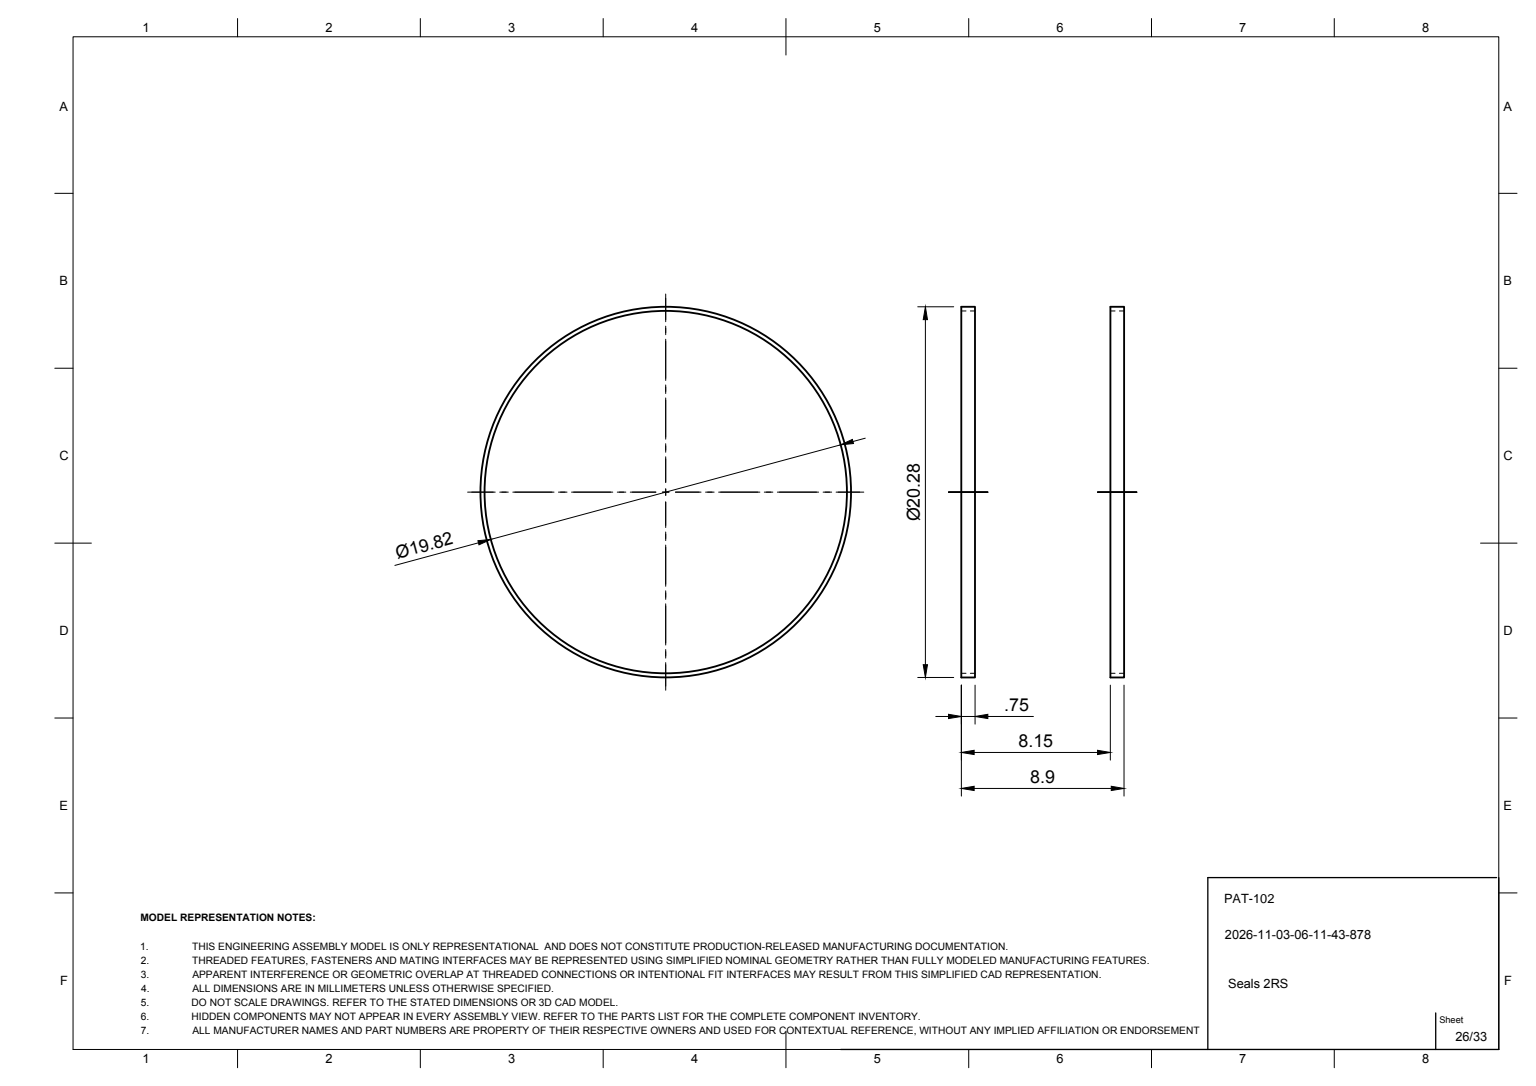
ISO-10303-21;
HEADER;
/* Generated by software containing ST-Developer
 * from STEP Tools, Inc. (www.steptools.com) 
 */

FILE_DESCRIPTION(
/* description */ ('Swing-away clamp arm'),
/* implementation_level */ '2;1');

FILE_NAME(
/* name */ 'Seals 2RS.step',
/* time_stamp */ '2026-10-28T03:26:03-07:00',
/* author */ (''),
/* organization */ (''),
/* preprocessor_version */ 'ST-DEVELOPER v20.2',
/* originating_system */ 'Autodesk Translation Framework v15.17.0.0',
/* authorisation */ '');

FILE_SCHEMA (('AUTOMOTIVE_DESIGN { 1 0 10303 214 3 1 1 }'));
ENDSEC;

DATA;
#10=MECHANICAL_DESIGN_GEOMETRIC_PRESENTATION_REPRESENTATION('',(#318,#319),#10627);
#259=SHAPE_REPRESENTATION_RELATIONSHIP('SRR','None',#10759,#285);
#285=ADVANCED_BREP_SHAPE_REPRESENTATION('',(#351,#352),#10618);
#318=STYLED_ITEM('',(#10965),#351);
#319=STYLED_ITEM('',(#10965),#352);
#351=MANIFOLD_SOLID_BREP('Body1',#4925);
#352=MANIFOLD_SOLID_BREP('Body2',#4926);
#437=FACE_BOUND('',#1253,.T.);
#438=FACE_BOUND('',#1256,.T.);
#439=FACE_BOUND('',#1259,.T.);
#440=FACE_BOUND('',#1262,.T.);
#591=PLANE('',#5692);
#592=PLANE('',#5697);
#593=PLANE('',#5700);
#594=PLANE('',#5705);
#866=FACE_OUTER_BOUND('',#1252,.T.);
#867=FACE_OUTER_BOUND('',#1254,.T.);
#868=FACE_OUTER_BOUND('',#1255,.T.);
#869=FACE_OUTER_BOUND('',#1257,.T.);
#870=FACE_OUTER_BOUND('',#1258,.T.);
#871=FACE_OUTER_BOUND('',#1260,.T.);
#872=FACE_OUTER_BOUND('',#1261,.T.);
#873=FACE_OUTER_BOUND('',#1263,.T.);
#1252=EDGE_LOOP('',(#4229));
#1253=EDGE_LOOP('',(#4230));
#1254=EDGE_LOOP('',(#4231,#4232,#4233,#4234));
#1255=EDGE_LOOP('',(#4235));
#1256=EDGE_LOOP('',(#4236));
#1257=EDGE_LOOP('',(#4237,#4238,#4239,#4240));
#1258=EDGE_LOOP('',(#4241));
#1259=EDGE_LOOP('',(#4242));
#1260=EDGE_LOOP('',(#4243,#4244,#4245,#4246));
#1261=EDGE_LOOP('',(#4247));
#1262=EDGE_LOOP('',(#4248));
#1263=EDGE_LOOP('',(#4249,#4250,#4251,#4252));
#1598=LINE('',#10232,#1920);
#1599=LINE('',#10237,#1921);
#1600=LINE('',#10246,#1922);
#1601=LINE('',#10251,#1923);
#1920=VECTOR('',#7065,1.013815);
#1921=VECTOR('',#7072,0.991185);
#1922=VECTOR('',#7083,1.013815);
#1923=VECTOR('',#7090,0.991185);
#2203=CIRCLE('',#5693,1.013815);
#2204=CIRCLE('',#5694,0.991185);
#2205=CIRCLE('',#5696,1.013815);
#2206=CIRCLE('',#5698,0.991185);
#2207=CIRCLE('',#5701,1.013815);
#2208=CIRCLE('',#5702,0.991185);
#2209=CIRCLE('',#5704,1.013815);
#2210=CIRCLE('',#5706,0.991185);
#2586=VERTEX_POINT('',#10225);
#2587=VERTEX_POINT('',#10227);
#2588=VERTEX_POINT('',#10230);
#2589=VERTEX_POINT('',#10234);
#2590=VERTEX_POINT('',#10239);
#2591=VERTEX_POINT('',#10241);
#2592=VERTEX_POINT('',#10244);
#2593=VERTEX_POINT('',#10248);
#3147=EDGE_CURVE('',#2586,#2586,#2203,.T.);
#3148=EDGE_CURVE('',#2587,#2587,#2204,.T.);
#3149=EDGE_CURVE('',#2588,#2588,#2205,.T.);
#3150=EDGE_CURVE('',#2588,#2586,#1598,.T.);
#3151=EDGE_CURVE('',#2589,#2589,#2206,.T.);
#3152=EDGE_CURVE('',#2589,#2587,#1599,.T.);
#3153=EDGE_CURVE('',#2590,#2590,#2207,.T.);
#3154=EDGE_CURVE('',#2591,#2591,#2208,.T.);
#3155=EDGE_CURVE('',#2592,#2592,#2209,.T.);
#3156=EDGE_CURVE('',#2592,#2590,#1600,.T.);
#3157=EDGE_CURVE('',#2593,#2593,#2210,.T.);
#3158=EDGE_CURVE('',#2593,#2591,#1601,.T.);
#4229=ORIENTED_EDGE('',*,*,#3147,.F.);
#4230=ORIENTED_EDGE('',*,*,#3148,.T.);
#4231=ORIENTED_EDGE('',*,*,#3149,.F.);
#4232=ORIENTED_EDGE('',*,*,#3150,.T.);
#4233=ORIENTED_EDGE('',*,*,#3147,.T.);
#4234=ORIENTED_EDGE('',*,*,#3150,.F.);
#4235=ORIENTED_EDGE('',*,*,#3149,.T.);
#4236=ORIENTED_EDGE('',*,*,#3151,.F.);
#4237=ORIENTED_EDGE('',*,*,#3151,.T.);
#4238=ORIENTED_EDGE('',*,*,#3152,.T.);
#4239=ORIENTED_EDGE('',*,*,#3148,.F.);
#4240=ORIENTED_EDGE('',*,*,#3152,.F.);
#4241=ORIENTED_EDGE('',*,*,#3153,.F.);
#4242=ORIENTED_EDGE('',*,*,#3154,.T.);
#4243=ORIENTED_EDGE('',*,*,#3155,.F.);
#4244=ORIENTED_EDGE('',*,*,#3156,.T.);
#4245=ORIENTED_EDGE('',*,*,#3153,.T.);
#4246=ORIENTED_EDGE('',*,*,#3156,.F.);
#4247=ORIENTED_EDGE('',*,*,#3155,.T.);
#4248=ORIENTED_EDGE('',*,*,#3157,.F.);
#4249=ORIENTED_EDGE('',*,*,#3157,.T.);
#4250=ORIENTED_EDGE('',*,*,#3158,.T.);
#4251=ORIENTED_EDGE('',*,*,#3154,.F.);
#4252=ORIENTED_EDGE('',*,*,#3158,.F.);
#4567=CYLINDRICAL_SURFACE('',#5695,1.013815);
#4568=CYLINDRICAL_SURFACE('',#5699,0.991185);
#4569=CYLINDRICAL_SURFACE('',#5703,1.013815);
#4570=CYLINDRICAL_SURFACE('',#5707,0.991185);
#4821=ADVANCED_FACE('',(#866,#437),#591,.T.);
#4822=ADVANCED_FACE('',(#867),#4567,.T.);
#4823=ADVANCED_FACE('',(#868,#438),#592,.T.);
#4824=ADVANCED_FACE('',(#869),#4568,.F.);
#4825=ADVANCED_FACE('',(#870,#439),#593,.T.);
#4826=ADVANCED_FACE('',(#871),#4569,.T.);
#4827=ADVANCED_FACE('',(#872,#440),#594,.T.);
#4828=ADVANCED_FACE('',(#873),#4570,.F.);
#4925=CLOSED_SHELL('',(#4821,#4822,#4823,#4824));
#4926=CLOSED_SHELL('',(#4825,#4826,#4827,#4828));
#5691=AXIS2_PLACEMENT_3D('',#10223,#7053,#7054);
#5692=AXIS2_PLACEMENT_3D('',#10224,#7055,#7056);
#5693=AXIS2_PLACEMENT_3D('',#10226,#7057,#7058);
#5694=AXIS2_PLACEMENT_3D('',#10228,#7059,#7060);
#5695=AXIS2_PLACEMENT_3D('',#10229,#7061,#7062);
#5696=AXIS2_PLACEMENT_3D('',#10231,#7063,#7064);
#5697=AXIS2_PLACEMENT_3D('',#10233,#7066,#7067);
#5698=AXIS2_PLACEMENT_3D('',#10235,#7068,#7069);
#5699=AXIS2_PLACEMENT_3D('',#10236,#7070,#7071);
#5700=AXIS2_PLACEMENT_3D('',#10238,#7073,#7074);
#5701=AXIS2_PLACEMENT_3D('',#10240,#7075,#7076);
#5702=AXIS2_PLACEMENT_3D('',#10242,#7077,#7078);
#5703=AXIS2_PLACEMENT_3D('',#10243,#7079,#7080);
#5704=AXIS2_PLACEMENT_3D('',#10245,#7081,#7082);
#5705=AXIS2_PLACEMENT_3D('',#10247,#7084,#7085);
#5706=AXIS2_PLACEMENT_3D('',#10249,#7086,#7087);
#5707=AXIS2_PLACEMENT_3D('',#10250,#7088,#7089);
#7053=DIRECTION('axis',(0.,0.,1.));
#7054=DIRECTION('refdir',(1.,0.,0.));
#7055=DIRECTION('center_axis',(0.,1.,0.));
#7056=DIRECTION('ref_axis',(0.,0.,1.));
#7057=DIRECTION('center_axis',(0.,-1.,0.));
#7058=DIRECTION('ref_axis',(1.,0.,0.));
#7059=DIRECTION('center_axis',(0.,-1.,0.));
#7060=DIRECTION('ref_axis',(1.,0.,0.));
#7061=DIRECTION('center_axis',(0.,-1.,0.));
#7062=DIRECTION('ref_axis',(1.,0.,0.));
#7063=DIRECTION('center_axis',(0.,-1.,0.));
#7064=DIRECTION('ref_axis',(1.,0.,0.));
#7065=DIRECTION('',(0.,1.,0.));
#7066=DIRECTION('center_axis',(0.,-1.,0.));
#7067=DIRECTION('ref_axis',(0.,0.,-1.));
#7068=DIRECTION('center_axis',(0.,-1.,0.));
#7069=DIRECTION('ref_axis',(1.,0.,0.));
#7070=DIRECTION('center_axis',(0.,-1.,0.));
#7071=DIRECTION('ref_axis',(1.,0.,0.));
#7072=DIRECTION('',(0.,1.,0.));
#7073=DIRECTION('center_axis',(0.,1.,0.));
#7074=DIRECTION('ref_axis',(0.,0.,1.));
#7075=DIRECTION('center_axis',(0.,-1.,0.));
#7076=DIRECTION('ref_axis',(1.,0.,0.));
#7077=DIRECTION('center_axis',(0.,-1.,0.));
#7078=DIRECTION('ref_axis',(1.,0.,0.));
#7079=DIRECTION('center_axis',(0.,-1.,0.));
#7080=DIRECTION('ref_axis',(1.,0.,0.));
#7081=DIRECTION('center_axis',(0.,-1.,0.));
#7082=DIRECTION('ref_axis',(1.,0.,0.));
#7083=DIRECTION('',(0.,1.,0.));
#7084=DIRECTION('center_axis',(0.,-1.,0.));
#7085=DIRECTION('ref_axis',(0.,0.,-1.));
#7086=DIRECTION('center_axis',(0.,-1.,0.));
#7087=DIRECTION('ref_axis',(1.,0.,0.));
#7088=DIRECTION('center_axis',(0.,-1.,0.));
#7089=DIRECTION('ref_axis',(1.,0.,0.));
#7090=DIRECTION('',(0.,1.,0.));
#10223=CARTESIAN_POINT('',(0.,0.,0.));
#10224=CARTESIAN_POINT('Origin',(1.013815,0.445,0.));
#10225=CARTESIAN_POINT('',(-1.013815,0.445,-1.24156529467757E-16));
#10226=CARTESIAN_POINT('Origin',(0.,0.445,0.));
#10227=CARTESIAN_POINT('',(-0.991185,0.445,-1.21385153761287E-16));
#10228=CARTESIAN_POINT('Origin',(0.,0.445,0.));
#10229=CARTESIAN_POINT('Origin',(0.,0.4075,0.));
#10230=CARTESIAN_POINT('',(-1.013815,0.37,-1.24156529467757E-16));
#10231=CARTESIAN_POINT('Origin',(0.,0.37,0.));
#10232=CARTESIAN_POINT('',(-1.013815,0.4075,-1.24156529467757E-16));
#10233=CARTESIAN_POINT('Origin',(0.991185,0.37,0.));
#10234=CARTESIAN_POINT('',(-0.991185,0.37,-1.21385153761287E-16));
#10235=CARTESIAN_POINT('Origin',(0.,0.37,0.));
#10236=CARTESIAN_POINT('Origin',(0.,0.4075,0.));
#10237=CARTESIAN_POINT('',(-0.991185,0.4075,-1.21385153761287E-16));
#10238=CARTESIAN_POINT('Origin',(1.013815,-0.37,0.));
#10239=CARTESIAN_POINT('',(-1.013815,-0.37,-1.24156529467757E-16));
#10240=CARTESIAN_POINT('Origin',(0.,-0.37,0.));
#10241=CARTESIAN_POINT('',(-0.991185,-0.37,-1.21385153761287E-16));
#10242=CARTESIAN_POINT('Origin',(0.,-0.37,0.));
#10243=CARTESIAN_POINT('Origin',(0.,-0.4075,0.));
#10244=CARTESIAN_POINT('',(-1.013815,-0.445,-1.24156529467757E-16));
#10245=CARTESIAN_POINT('Origin',(0.,-0.445,0.));
#10246=CARTESIAN_POINT('',(-1.013815,-0.4075,-1.24156529467757E-16));
#10247=CARTESIAN_POINT('Origin',(0.991185,-0.445,0.));
#10248=CARTESIAN_POINT('',(-0.991185,-0.445,-1.21385153761287E-16));
#10249=CARTESIAN_POINT('Origin',(0.,-0.445,0.));
#10250=CARTESIAN_POINT('Origin',(0.,-0.4075,0.));
#10251=CARTESIAN_POINT('',(-0.991185,-0.4075,-1.21385153761287E-16));
#10586=UNCERTAINTY_MEASURE_WITH_UNIT(LENGTH_MEASURE(0.001),#10628,
'DISTANCE_ACCURACY_VALUE',
'Maximum model space distance between geometric entities at asserted c
onnectivities');
#10595=UNCERTAINTY_MEASURE_WITH_UNIT(LENGTH_MEASURE(0.001),#10628,
'DISTANCE_ACCURACY_VALUE',
'Maximum model space distance between geometric entities at asserted c
onnectivities');
#10618=(
GEOMETRIC_REPRESENTATION_CONTEXT(3)
GLOBAL_UNCERTAINTY_ASSIGNED_CONTEXT((#10586))
GLOBAL_UNIT_ASSIGNED_CONTEXT((#10628,#10630,#10631))
REPRESENTATION_CONTEXT('','3D')
);
#10627=(
GEOMETRIC_REPRESENTATION_CONTEXT(3)
GLOBAL_UNCERTAINTY_ASSIGNED_CONTEXT((#10595))
GLOBAL_UNIT_ASSIGNED_CONTEXT((#10628,#10630,#10631))
REPRESENTATION_CONTEXT('','3D')
);
#10628=(
LENGTH_UNIT()
NAMED_UNIT(*)
SI_UNIT(.CENTI.,.METRE.)
);
#10630=(
NAMED_UNIT(*)
PLANE_ANGLE_UNIT()
SI_UNIT($,.RADIAN.)
);
#10631=(
NAMED_UNIT(*)
SI_UNIT($,.STERADIAN.)
SOLID_ANGLE_UNIT()
);
#10654=SHAPE_DEFINITION_REPRESENTATION(#10695,#10759);
#10695=PRODUCT_DEFINITION_SHAPE('',$,#10791);
#10759=SHAPE_REPRESENTATION('',(#5691),#10618);
#10768=PRODUCT_DEFINITION_CONTEXT('part definition',#10863,'design');
#10791=PRODUCT_DEFINITION('Seals 2RS','Seals 2RS',#10822,#10768);
#10822=PRODUCT_DEFINITION_FORMATION('',$,#10887);
#10863=APPLICATION_CONTEXT(
'Core Data for Automotive Mechanical Design Process');
#10864=PRODUCT_CONTEXT('part definition',#10863,'mechanical');
#10887=PRODUCT('Seals 2RS','Seals 2RS','Seals 2RS',(#10864));
#10959=COLOUR_RGB('Grey',0.48,0.52,0.57);
#10960=FILL_AREA_STYLE_COLOUR('',#10959);
#10961=FILL_AREA_STYLE('',(#10960));
#10962=SURFACE_STYLE_FILL_AREA(#10961);
#10963=SURFACE_SIDE_STYLE('',(#10962));
#10964=SURFACE_STYLE_USAGE(.BOTH.,#10963);
#10965=PRESENTATION_STYLE_ASSIGNMENT((#10964));
ENDSEC;
END-ISO-10303-21;
